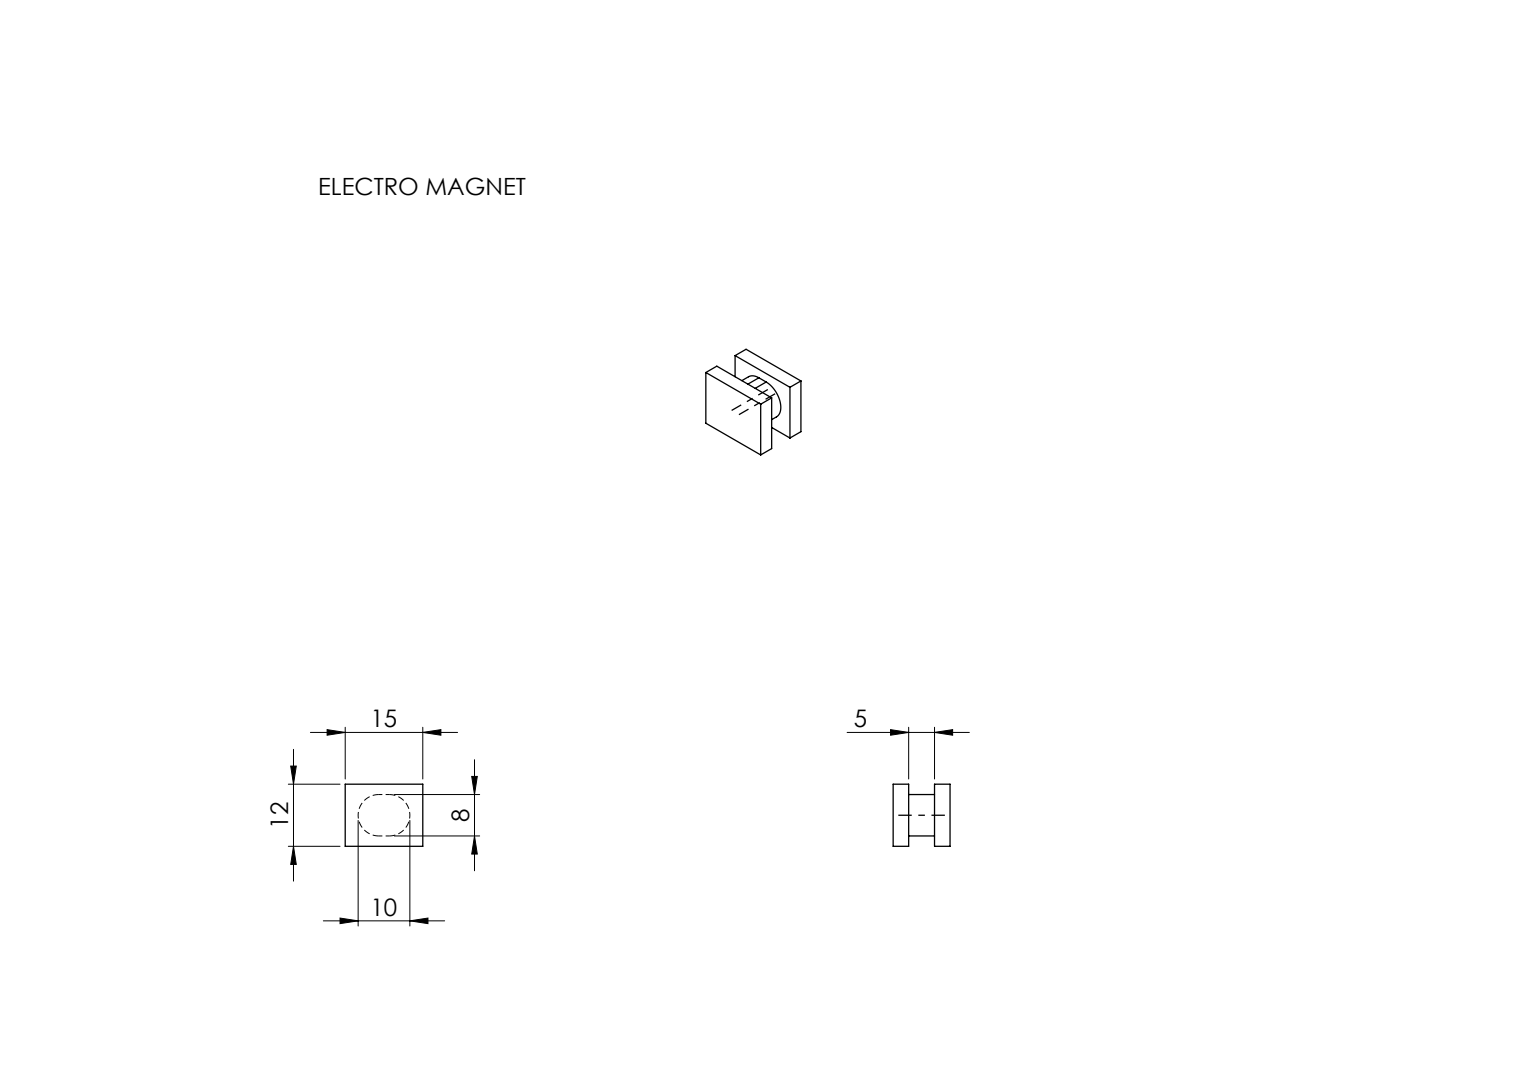
ISO-10303-21;
HEADER;
FILE_DESCRIPTION (('STEP AP214'),
    '1' );
FILE_NAME ('electro magnet.step',
    '2026-10-08T14:41:38',
    ( '' ),
    ( '' ),
    'SwSTEP 2.0',
    'SolidWorks 2026',
    '' );
FILE_SCHEMA (( 'AUTOMOTIVE_DESIGN' ));
ENDSEC;

DATA;
#101=ORIENTED_EDGE ( 'NONE', *, *, #16409, .T. ) ;
#145=VECTOR ( 'NONE', #11392, 1000.000000000000000 ) ;
#171=( NAMED_UNIT ( * ) SI_UNIT ( $, .STERADIAN. ) SOLID_ANGLE_UNIT ( ) );
#187=LINE ( 'NONE', #12134, #5316 ) ;
#194=FACE_OUTER_BOUND ( 'NONE', #3643, .T. ) ;
#207=CIRCLE ( 'NONE', #14282, 4.000000000000001776 ) ;
#299=AXIS2_PLACEMENT_3D ( 'NONE', #12287, #10903, #18180 ) ;
#302=ADVANCED_FACE ( 'NONE', ( #4804 ), #6459, .T. ) ;
#408=LINE ( 'NONE', #5209, #9039 ) ;
#421=UNCERTAINTY_MEASURE_WITH_UNIT (LENGTH_MEASURE( 1.000000000000000082E-05 ), #7921, 'distance_accuracy_value', 'NONE');
#477=EDGE_CURVE ( 'NONE', #3996, #8594, #18791, .T. ) ;
#486=VECTOR ( 'NONE', #10587, 1000.000000000000000 ) ;
#516=VECTOR ( 'NONE', #18188, 1000.000000000000000 ) ;
#549=SURFACE_STYLE_FILL_AREA ( #12311 ) ;
#556=ORIENTED_EDGE ( 'NONE', *, *, #4978, .F. ) ;
#594=CIRCLE ( 'NONE', #10600, 4.000000000000001776 ) ;
#694=ORIENTED_EDGE ( 'NONE', *, *, #13084, .T. ) ;
#703=AXIS2_PLACEMENT_3D ( 'NONE', #5641, #5740, #11602 ) ;
#724=PLANE ( 'NONE',  #16794 ) ;
#781=ADVANCED_FACE ( 'NONE', ( #18300 ), #17023, .F. ) ;
#858=ORIENTED_EDGE ( 'NONE', *, *, #9631, .T. ) ;
#920=CARTESIAN_POINT ( 'NONE',  ( -0.9999999999999945599, -28.00000000000000000, 9.500000000000001776 ) ) ;
#936=AXIS2_PLACEMENT_3D ( 'NONE', #14392, #3821, #15873 ) ;
#1085=ORIENTED_EDGE ( 'NONE', *, *, #13084, .F. ) ;
#1145=ORIENTED_EDGE ( 'NONE', *, *, #7309, .F. ) ;
#1159=LINE ( 'NONE', #17905, #8587 ) ;
#1304=ORIENTED_EDGE ( 'NONE', *, *, #4606, .F. ) ;
#1306=VECTOR ( 'NONE', #7410, 1000.000000000000000 ) ;
#1365=PLANE ( 'NONE',  #2180 ) ;
#1395=CARTESIAN_POINT ( 'NONE',  ( -0.9999999999999945599, -32.00000000000000000, 4.500000000000000888 ) ) ;
#1406=LINE ( 'NONE', #6021, #14690 ) ;
#1438=DIRECTION ( 'NONE',  ( 2.312964634635742957E-16, -1.000000000000000000, 0.000000000000000000 ) ) ;
#1483=ORIENTED_EDGE ( 'NONE', *, *, #18646, .T. ) ;
#1497=DIRECTION ( 'NONE',  ( -1.000000000000000000, 0.000000000000000000, 0.000000000000000000 ) ) ;
#1502=ADVANCED_FACE ( 'NONE', ( #11641 ), #1365, .F. ) ;
#1513=DIRECTION ( 'NONE',  ( -0.000000000000000000, -0.000000000000000000, -1.000000000000000000 ) ) ;
#1536=CARTESIAN_POINT ( 'NONE',  ( -0.9999999999999945599, -28.00000000000000000, 9.500000000000001776 ) ) ;
#1537=DIRECTION ( 'NONE',  ( -0.000000000000000000, -0.000000000000000000, -1.000000000000000000 ) ) ;
#1592=CARTESIAN_POINT ( 'NONE',  ( -0.9999999999999945599, -28.00000000000000000, 9.500000000000001776 ) ) ;
#1613=VECTOR ( 'NONE', #1909, 1000.000000000000000 ) ;
#1632=EDGE_CURVE ( 'NONE', #10157, #8595, #9199, .T. ) ;
#1643=CARTESIAN_POINT ( 'NONE',  ( 7.500000000000005329, -38.00000000000000000, 9.500000000000001776 ) ) ;
#1698=CARTESIAN_POINT ( 'NONE',  ( 1.000000000000000222, -28.00000000000000000, 9.500000000000001776 ) ) ;
#1719=EDGE_CURVE ( 'NONE', #7260, #9088, #15187, .T. ) ;
#1757=DIRECTION ( 'NONE',  ( -1.000000000000000000, 0.000000000000000000, 0.000000000000000000 ) ) ;
#1761=EDGE_CURVE ( 'NONE', #16018, #13407, #187, .T. ) ;
#1781=DIRECTION ( 'NONE',  ( 0.000000000000000000, -1.000000000000000000, 0.000000000000000000 ) ) ;
#1791=AXIS2_PLACEMENT_3D ( 'NONE', #13713, #4815, #7646 ) ;
#1807=CARTESIAN_POINT ( 'NONE',  ( 7.500000000000005329, -26.00000000000000000, 12.50000000000000000 ) ) ;
#1820=EDGE_CURVE ( 'NONE', #6791, #1960, #10951, .T. ) ;
#1857=EDGE_LOOP ( 'NONE', ( #12020, #9397, #15224, #9214 ) ) ;
#1909=DIRECTION ( 'NONE',  ( -0.000000000000000000, -0.000000000000000000, -1.000000000000000000 ) ) ;
#1960=VERTEX_POINT ( 'NONE', #3801 ) ;
#2012=DIRECTION ( 'NONE',  ( -1.000000000000000000, -2.312964634635742957E-16, 0.000000000000000000 ) ) ;
#2145=ORIENTED_EDGE ( 'NONE', *, *, #1820, .F. ) ;
#2180=AXIS2_PLACEMENT_3D ( 'NONE', #8702, #9970, #15972 ) ;
#2370=AXIS2_PLACEMENT_3D ( 'NONE', #8705, #13017, #9888 ) ;
#2375=CARTESIAN_POINT ( 'NONE',  ( 1.000000000000001332, -36.00000000000000711, 4.500000000000000888 ) ) ;
#2397=ADVANCED_FACE ( 'NONE', ( #5068 ), #3299, .F. ) ;
#2504=CARTESIAN_POINT ( 'NONE',  ( 7.500000000000005329, -38.00000000000000000, 4.500000000000000888 ) ) ;
#2546=VECTOR ( 'NONE', #1781, 1000.000000000000000 ) ;
#2553=ORIENTED_EDGE ( 'NONE', *, *, #18646, .F. ) ;
#2695=CIRCLE ( 'NONE', #18053, 4.000000000000001776 ) ;
#2770=FACE_OUTER_BOUND ( 'NONE', #13066, .T. ) ;
#2903=CARTESIAN_POINT ( 'NONE',  ( 7.500000000000005329, -26.00000000000000000, 12.50000000000000000 ) ) ;
#2954=DIRECTION ( 'NONE',  ( -0.000000000000000000, -0.000000000000000000, -1.000000000000000000 ) ) ;
#2987=DIRECTION ( 'NONE',  ( -0.000000000000000000, -0.000000000000000000, -1.000000000000000000 ) ) ;
#3004=VECTOR ( 'NONE', #4487, 1000.000000000000000 ) ;
#3066=VERTEX_POINT ( 'NONE', #15868 ) ;
#3093=DIRECTION ( 'NONE',  ( 0.000000000000000000, -0.000000000000000000, -1.000000000000000000 ) ) ;
#3134=ORIENTED_EDGE ( 'NONE', *, *, #15716, .T. ) ;
#3138=LINE ( 'NONE', #14011, #12507 ) ;
#3168=EDGE_LOOP ( 'NONE', ( #11221, #15374, #4325, #14700 ) ) ;
#3210=SURFACE_STYLE_USAGE ( .BOTH. , #13686 ) ;
#3228=FACE_OUTER_BOUND ( 'NONE', #8260, .T. ) ;
#3299=PLANE ( 'NONE',  #14340 ) ;
#3319=ORIENTED_EDGE ( 'NONE', *, *, #4999, .F. ) ;
#3418=EDGE_CURVE ( 'NONE', #4550, #8057, #11780, .T. ) ;
#3419=DIRECTION ( 'NONE',  ( 0.000000000000000000, 1.000000000000000000, -0.000000000000000000 ) ) ;
#3467=FACE_OUTER_BOUND ( 'NONE', #17184, .T. ) ;
#3512=ORIENTED_EDGE ( 'NONE', *, *, #10326, .F. ) ;
#3516=DIRECTION ( 'NONE',  ( -0.000000000000000000, -0.000000000000000000, -1.000000000000000000 ) ) ;
#3583=DIRECTION ( 'NONE',  ( 0.000000000000000000, 1.000000000000000000, 0.000000000000000000 ) ) ;
#3585=( NAMED_UNIT ( * ) SI_UNIT ( $, .STERADIAN. ) SOLID_ANGLE_UNIT ( ) );
#3620=ORIENTED_EDGE ( 'NONE', *, *, #9152, .T. ) ;
#3643=EDGE_LOOP ( 'NONE', ( #7791, #3319, #1304, #15009 ) ) ;
#3801=CARTESIAN_POINT ( 'NONE',  ( 7.500000000000005329, -38.00000000000000000, 9.500000000000001776 ) ) ;
#3821=DIRECTION ( 'NONE',  ( 0.000000000000000000, 0.000000000000000000, 1.000000000000000000 ) ) ;
#3830=CARTESIAN_POINT ( 'NONE',  ( 7.500000000000005329, -26.00000000000000000, 9.500000000000001776 ) ) ;
#3996=VERTEX_POINT ( 'NONE', #10683 ) ;
#4016=ORIENTED_EDGE ( 'NONE', *, *, #1632, .F. ) ;
#4029=EDGE_CURVE ( 'NONE', #6116, #3066, #10772, .T. ) ;
#4099=CIRCLE ( 'NONE', #8479, 4.000000000000001776 ) ;
#4143=DIRECTION ( 'NONE',  ( -1.000000000000000000, -0.000000000000000000, -0.000000000000000000 ) ) ;
#4193=ORIENTED_EDGE ( 'NONE', *, *, #4980, .T. ) ;
#4287=LINE ( 'NONE', #16045, #3004 ) ;
#4297=DIRECTION ( 'NONE',  ( 0.000000000000000000, -0.000000000000000000, 1.000000000000000000 ) ) ;
#4325=ORIENTED_EDGE ( 'NONE', *, *, #9152, .F. ) ;
#4341=UNCERTAINTY_MEASURE_WITH_UNIT (LENGTH_MEASURE( 1.000000000000000082E-05 ), #4793, 'distance_accuracy_value', 'NONE');
#4347=CARTESIAN_POINT ( 'NONE',  ( -7.499999999999994671, -38.00000000000000000, 4.500000000000000888 ) ) ;
#4417=VECTOR ( 'NONE', #15037, 1000.000000000000000 ) ;
#4484=LINE ( 'NONE', #1643, #5058 ) ;
#4487=DIRECTION ( 'NONE',  ( -0.000000000000000000, -0.000000000000000000, -1.000000000000000000 ) ) ;
#4537=VECTOR ( 'NONE', #6993, 1000.000000000000000 ) ;
#4550=VERTEX_POINT ( 'NONE', #13696 ) ;
#4606=EDGE_CURVE ( 'NONE', #4550, #3996, #12892, .T. ) ;
#4642=DIRECTION ( 'NONE',  ( 0.000000000000000000, 0.000000000000000000, 1.000000000000000000 ) ) ;
#4676=DIRECTION ( 'NONE',  ( 0.000000000000000000, 1.000000000000000000, 0.000000000000000000 ) ) ;
#4677=LINE ( 'NONE', #2903, #12097 ) ;
#4736=CARTESIAN_POINT ( 'NONE',  ( -0.9999999999999945599, -28.00000000000000000, 4.500000000000000888 ) ) ;
#4754=ORIENTED_EDGE ( 'NONE', *, *, #15964, .F. ) ;
#4780=DIRECTION ( 'NONE',  ( 1.000000000000000000, 2.312964634635742957E-16, 0.000000000000000000 ) ) ;
#4793=( LENGTH_UNIT ( ) NAMED_UNIT ( * ) SI_UNIT ( .MILLI., .METRE. ) );
#4804=FACE_OUTER_BOUND ( 'NONE', #13698, .T. ) ;
#4815=DIRECTION ( 'NONE',  ( 0.000000000000000000, 0.000000000000000000, 1.000000000000000000 ) ) ;
#4856=CARTESIAN_POINT ( 'NONE',  ( -0.9999999999999945599, -36.00000000000000711, 9.500000000000001776 ) ) ;
#4861=VECTOR ( 'NONE', #6043, 1000.000000000000000 ) ;
#4937=DIRECTION ( 'NONE',  ( 1.000000000000000000, 0.000000000000000000, 0.000000000000000000 ) ) ;
#4949=FACE_BOUND ( 'NONE', #8943, .T. ) ;
#4978=EDGE_CURVE ( 'NONE', #8057, #16018, #408, .T. ) ;
#4980=EDGE_CURVE ( 'NONE', #3066, #10268, #594, .T. ) ;
#4999=EDGE_CURVE ( 'NONE', #3996, #16018, #18552, .T. ) ;
#5058=VECTOR ( 'NONE', #17914, 1000.000000000000000 ) ;
#5068=FACE_OUTER_BOUND ( 'NONE', #10560, .T. ) ;
#5071=SURFACE_SIDE_STYLE ('',( #549 ) ) ;
#5100=ORIENTED_EDGE ( 'NONE', *, *, #13421, .T. ) ;
#5175=DIRECTION ( 'NONE',  ( 1.000000000000000000, -0.000000000000000000, -0.000000000000000000 ) ) ;
#5179=CARTESIAN_POINT ( 'NONE',  ( -7.499999999999994671, -38.00000000000000000, 9.500000000000001776 ) ) ;
#5209=CARTESIAN_POINT ( 'NONE',  ( 7.500000000000005329, -38.00000000000000000, 1.500000000000000000 ) ) ;
#5256=FILL_AREA_STYLE_COLOUR ( '', #6784 ) ;
#5286=ORIENTED_EDGE ( 'NONE', *, *, #1820, .T. ) ;
#5292=ORIENTED_EDGE ( 'NONE', *, *, #7515, .F. ) ;
#5316=VECTOR ( 'NONE', #13700, 1000.000000000000000 ) ;
#5340=LINE ( 'NONE', #11587, #4537 ) ;
#5366=DIRECTION ( 'NONE',  ( 0.000000000000000000, 1.000000000000000000, 0.000000000000000000 ) ) ;
#5399=DIRECTION ( 'NONE',  ( -0.000000000000000000, -1.000000000000000000, -0.000000000000000000 ) ) ;
#5641=CARTESIAN_POINT ( 'NONE',  ( 0.000000000000000000, 0.000000000000000000, 4.500000000000000888 ) ) ;
#5740=DIRECTION ( 'NONE',  ( 0.000000000000000000, -0.000000000000000000, 1.000000000000000000 ) ) ;
#5768=ORIENTED_EDGE ( 'NONE', *, *, #14263, .F. ) ;
#5776=FACE_OUTER_BOUND ( 'NONE', #3168, .T. ) ;
#5801=PRODUCT_CONTEXT ( 'NONE', #9697, 'mechanical' ) ;
#5824=DIRECTION ( 'NONE',  ( -0.000000000000000000, -0.000000000000000000, -1.000000000000000000 ) ) ;
#5829=PRODUCT_DEFINITION_SHAPE ( 'NONE', 'NONE',  #16256 ) ;
#5848=CARTESIAN_POINT ( 'NONE',  ( -7.499999999999994671, -38.00000000000000000, 12.50000000000000000 ) ) ;
#5973=DIRECTION ( 'NONE',  ( -0.000000000000000000, -0.000000000000000000, -1.000000000000000000 ) ) ;
#6021=CARTESIAN_POINT ( 'NONE',  ( -7.499999999999994671, -26.00000000000000355, 9.500000000000001776 ) ) ;
#6043=DIRECTION ( 'NONE',  ( -1.000000000000000000, -2.312964634635742957E-16, 0.000000000000000000 ) ) ;
#6055=EDGE_CURVE ( 'NONE', #13407, #9088, #3138, .T. ) ;
#6116=VERTEX_POINT ( 'NONE', #9842 ) ;
#6117=DIRECTION ( 'NONE',  ( 0.000000000000000000, -0.000000000000000000, 1.000000000000000000 ) ) ;
#6153=ORIENTED_EDGE ( 'NONE', *, *, #7072, .F. ) ;
#6155=( NAMED_UNIT ( * ) PLANE_ANGLE_UNIT ( ) SI_UNIT ( $, .RADIAN. ) );
#6179=ADVANCED_FACE ( 'NONE', ( #2770 ), #7287, .F. ) ;
#6181=ORIENTED_EDGE ( 'NONE', *, *, #1761, .F. ) ;
#6195=DIRECTION ( 'NONE',  ( 1.000000000000000000, 0.000000000000000000, 0.000000000000000000 ) ) ;
#6201=LINE ( 'NONE', #7361, #486 ) ;
#6292=CARTESIAN_POINT ( 'NONE',  ( 7.500000000000005329, -26.00000000000000000, 4.500000000000000888 ) ) ;
#6314=VECTOR ( 'NONE', #4143, 1000.000000000000000 ) ;
#6324=CARTESIAN_POINT ( 'NONE',  ( -0.9999999999999945599, -36.00000000000000711, 4.500000000000000888 ) ) ;
#6328=UNCERTAINTY_MEASURE_WITH_UNIT (LENGTH_MEASURE( 1.000000000000000082E-05 ), #18306, 'distance_accuracy_value', 'NONE');
#6349=CLOSED_SHELL ( 'NONE', ( #17179, #14773, #17898, #14461, #9964, #10792, #11208, #6407, #6179, #302, #8220, #13820, #9503, #781, #1502, #2397, #18291 ) ) ;
#6354=FILL_AREA_STYLE_COLOUR ( '', #16103 ) ;
#6370=CARTESIAN_POINT ( 'NONE',  ( -0.9999999999999945599, -32.00000000000000000, 9.500000000000001776 ) ) ;
#6407=ADVANCED_FACE ( 'NONE', ( #13950 ), #9334, .T. ) ;
#6421=CARTESIAN_POINT ( 'NONE',  ( -7.499999999999994671, -26.00000000000000355, 12.50000000000000000 ) ) ;
#6422=CARTESIAN_POINT ( 'NONE',  ( -4.999999999999996447, -32.00000000000000000, 4.500000000000000888 ) ) ;
#6459=CYLINDRICAL_SURFACE ( 'NONE', #17272, 4.000000000000001776 ) ;
#6532=CARTESIAN_POINT ( 'NONE',  ( -7.499999999999994671, -38.00000000000000000, 12.50000000000000000 ) ) ;
#6568=VECTOR ( 'NONE', #7836, 1000.000000000000000 ) ;
#6618=ORIENTED_EDGE ( 'NONE', *, *, #11880, .F. ) ;
#6698=VERTEX_POINT ( 'NONE', #13234 ) ;
#6740=DIRECTION ( 'NONE',  ( 0.000000000000000000, 0.000000000000000000, 1.000000000000000000 ) ) ;
#6750=EDGE_LOOP ( 'NONE', ( #7814, #10770, #16833, #12425 ) ) ;
#6784=COLOUR_RGB ( '', 0.66274510, 0.83137255, 0.94901961) ;
#6791=VERTEX_POINT ( 'NONE', #7763 ) ;
#6796=MECHANICAL_DESIGN_GEOMETRIC_PRESENTATION_REPRESENTATION('',(#17732),#17748);
#6899=CARTESIAN_POINT ( 'NONE',  ( 7.500000000000005329, -26.00000000000000000, 1.500000000000000000 ) ) ;
#6941=CARTESIAN_POINT ( 'NONE',  ( 0.000000000000000000, 0.000000000000000000, 1.500000000000000000 ) ) ;
#6993=DIRECTION ( 'NONE',  ( 1.000000000000000000, 0.000000000000000000, 0.000000000000000000 ) ) ;
#6996=LINE ( 'NONE', #920, #15048 ) ;
#7009=FACE_OUTER_BOUND ( 'NONE', #12217, .T. ) ;
#7045=LINE ( 'NONE', #18826, #13144 ) ;
#7070=CARTESIAN_POINT ( 'NONE',  ( -0.9999999999999945599, -28.00000000000000000, 9.500000000000001776 ) ) ;
#7072=EDGE_CURVE ( 'NONE', #8851, #8886, #6996, .T. ) ;
#7107=FACE_BOUND ( 'NONE', #10188, .T. ) ;
#7146=ORIENTED_EDGE ( 'NONE', *, *, #12750, .F. ) ;
#7161=ORIENTED_EDGE ( 'NONE', *, *, #10010, .T. ) ;
#7165=DIRECTION ( 'NONE',  ( 0.000000000000000000, 0.000000000000000000, 1.000000000000000000 ) ) ;
#7183=DIRECTION ( 'NONE',  ( 0.000000000000000000, 1.000000000000000000, 0.000000000000000000 ) ) ;
#7213=FACE_OUTER_BOUND ( 'NONE', #12120, .T. ) ;
#7260=VERTEX_POINT ( 'NONE', #18182 ) ;
#7287=PLANE ( 'NONE',  #15329 ) ;
#7309=EDGE_CURVE ( 'NONE', #3066, #7522, #16707, .T. ) ;
#7361=CARTESIAN_POINT ( 'NONE',  ( -0.9999999999999945599, -28.00000000000000000, 4.500000000000000888 ) ) ;
#7382=DIRECTION ( 'NONE',  ( 0.000000000000000000, -1.000000000000000000, 0.000000000000000000 ) ) ;
#7410=DIRECTION ( 'NONE',  ( 1.000000000000000000, 0.000000000000000000, 0.000000000000000000 ) ) ;
#7424=CARTESIAN_POINT ( 'NONE',  ( 7.500000000000005329, -38.00000000000000000, 4.500000000000000888 ) ) ;
#7515=EDGE_CURVE ( 'NONE', #7522, #8981, #4099, .T. ) ;
#7522=VERTEX_POINT ( 'NONE', #2375 ) ;
#7543=ORIENTED_EDGE ( 'NONE', *, *, #7625, .F. ) ;
#7625=EDGE_CURVE ( 'NONE', #10268, #8851, #10191, .T. ) ;
#7646=DIRECTION ( 'NONE',  ( 1.000000000000000000, 0.000000000000000000, 0.000000000000000000 ) ) ;
#7678=DIRECTION ( 'NONE',  ( -0.000000000000000000, -0.000000000000000000, -1.000000000000000000 ) ) ;
#7763=CARTESIAN_POINT ( 'NONE',  ( -7.499999999999994671, -38.00000000000000000, 9.500000000000001776 ) ) ;
#7791=ORIENTED_EDGE ( 'NONE', *, *, #4978, .T. ) ;
#7799=LINE ( 'NONE', #16423, #4861 ) ;
#7814=ORIENTED_EDGE ( 'NONE', *, *, #6055, .T. ) ;
#7836=DIRECTION ( 'NONE',  ( 1.000000000000000000, 0.000000000000000000, 0.000000000000000000 ) ) ;
#7921=( LENGTH_UNIT ( ) NAMED_UNIT ( * ) SI_UNIT ( .MILLI., .METRE. ) );
#7939=DIRECTION ( 'NONE',  ( 1.000000000000000000, 0.000000000000000000, 0.000000000000000000 ) ) ;
#7941=DIRECTION ( 'NONE',  ( 0.000000000000000000, 0.000000000000000000, 1.000000000000000000 ) ) ;
#7996=VECTOR ( 'NONE', #2012, 1000.000000000000000 ) ;
#8057=VERTEX_POINT ( 'NONE', #18615 ) ;
#8205=VECTOR ( 'NONE', #4676, 1000.000000000000000 ) ;
#8220=ADVANCED_FACE ( 'NONE', ( #7213 ), #9075, .F. ) ;
#8254=EDGE_CURVE ( 'NONE', #15143, #13986, #10436, .T. ) ;
#8255=ORIENTED_EDGE ( 'NONE', *, *, #4029, .F. ) ;
#8260=EDGE_LOOP ( 'NONE', ( #7161, #17171, #11662, #12090 ) ) ;
#8398=EDGE_CURVE ( 'NONE', #13986, #10157, #16928, .T. ) ;
#8439=ORIENTED_EDGE ( 'NONE', *, *, #11905, .F. ) ;
#8479=AXIS2_PLACEMENT_3D ( 'NONE', #12850, #7165, #14425 ) ;
#8513=ORIENTED_EDGE ( 'NONE', *, *, #11880, .T. ) ;
#8587=VECTOR ( 'NONE', #2987, 1000.000000000000000 ) ;
#8594=VERTEX_POINT ( 'NONE', #12688 ) ;
#8595=VERTEX_POINT ( 'NONE', #17659 ) ;
#8702=CARTESIAN_POINT ( 'NONE',  ( -7.499999999999994671, -26.00000000000000355, 12.50000000000000000 ) ) ;
#8705=CARTESIAN_POINT ( 'NONE',  ( -7.499999999999994671, -38.00000000000000000, 4.500000000000000888 ) ) ;
#8730=CYLINDRICAL_SURFACE ( 'NONE', #11736, 4.000000000000001776 ) ;
#8843=PRODUCT_DEFINITION_CONTEXT ( 'detailed design', #13441, 'design' ) ;
#8851=VERTEX_POINT ( 'NONE', #1592 ) ;
#8886=VERTEX_POINT ( 'NONE', #4736 ) ;
#8889=PLANE ( 'NONE',  #19275 ) ;
#8900=EDGE_LOOP ( 'NONE', ( #19185, #10269, #3512, #12152 ) ) ;
#8905=CARTESIAN_POINT ( 'NONE',  ( 7.500000000000005329, -38.00000000000000000, 12.50000000000000000 ) ) ;
#8943=EDGE_LOOP ( 'NONE', ( #16290, #1483, #858, #18898, #4193 ) ) ;
#8981=VERTEX_POINT ( 'NONE', #17077 ) ;
#9039=VECTOR ( 'NONE', #11165, 1000.000000000000000 ) ;
#9075=PLANE ( 'NONE',  #11609 ) ;
#9088=VERTEX_POINT ( 'NONE', #18360 ) ;
#9152=EDGE_CURVE ( 'NONE', #7260, #4550, #7045, .T. ) ;
#9157=LINE ( 'NONE', #6421, #1613 ) ;
#9199=LINE ( 'NONE', #18127, #14073 ) ;
#9214=ORIENTED_EDGE ( 'NONE', *, *, #15716, .F. ) ;
#9240=AXIS2_PLACEMENT_3D ( 'NONE', #15325, #9628, #18669 ) ;
#9318=CARTESIAN_POINT ( 'NONE',  ( 7.500000000000005329, -38.00000000000000000, 4.500000000000000888 ) ) ;
#9323=CARTESIAN_POINT ( 'NONE',  ( 7.500000000000005329, -38.00000000000000000, 1.500000000000000000 ) ) ;
#9334=CYLINDRICAL_SURFACE ( 'NONE', #299, 4.000000000000001776 ) ;
#9369=( NAMED_UNIT ( * ) PLANE_ANGLE_UNIT ( ) SI_UNIT ( $, .RADIAN. ) );
#9397=ORIENTED_EDGE ( 'NONE', *, *, #15964, .T. ) ;
#9483=DIRECTION ( 'NONE',  ( -1.000000000000000000, 0.000000000000000000, 0.000000000000000000 ) ) ;
#9503=ADVANCED_FACE ( 'NONE', ( #3228 ), #15189, .F. ) ;
#9628=DIRECTION ( 'NONE',  ( 0.000000000000000000, -0.000000000000000000, 1.000000000000000000 ) ) ;
#9631=EDGE_CURVE ( 'NONE', #11032, #6116, #11288, .T. ) ;
#9684=ORIENTED_EDGE ( 'NONE', *, *, #477, .T. ) ;
#9697=APPLICATION_CONTEXT ( 'automotive_design' ) ;
#9737=VECTOR ( 'NONE', #13830, 1000.000000000000000 ) ;
#9840=ORIENTED_EDGE ( 'NONE', *, *, #10010, .F. ) ;
#9842=CARTESIAN_POINT ( 'NONE',  ( -0.9999999999999945599, -36.00000000000000711, 9.500000000000001776 ) ) ;
#9864=ORIENTED_EDGE ( 'NONE', *, *, #18143, .F. ) ;
#9872=FACE_OUTER_BOUND ( 'NONE', #18837, .T. ) ;
#9888=DIRECTION ( 'NONE',  ( 0.000000000000000000, 0.000000000000000000, -1.000000000000000000 ) ) ;
#9897=VECTOR ( 'NONE', #2954, 1000.000000000000000 ) ;
#9964=ADVANCED_FACE ( 'NONE', ( #13279 ), #19376, .F. ) ;
#9970=DIRECTION ( 'NONE',  ( 1.000000000000000000, 0.000000000000000000, -0.000000000000000000 ) ) ;
#9978=ORIENTED_EDGE ( 'NONE', *, *, #13207, .T. ) ;
#10010=EDGE_CURVE ( 'NONE', #1960, #14775, #4484, .T. ) ;
#10089=VERTEX_POINT ( 'NONE', #6324 ) ;
#10101=EDGE_CURVE ( 'NONE', #8595, #6698, #9157, .T. ) ;
#10157=VERTEX_POINT ( 'NONE', #1807 ) ;
#10188=EDGE_LOOP ( 'NONE', ( #18902, #5768, #5292, #11263, #7146 ) ) ;
#10191=LINE ( 'NONE', #7070, #6314 ) ;
#10268=VERTEX_POINT ( 'NONE', #15592 ) ;
#10269=ORIENTED_EDGE ( 'NONE', *, *, #13095, .F. ) ;
#10310=EDGE_CURVE ( 'NONE', #8594, #13407, #10880, .T. ) ;
#10326=EDGE_CURVE ( 'NONE', #8595, #15143, #18551, .T. ) ;
#10436=LINE ( 'NONE', #5848, #1306 ) ;
#10511=CARTESIAN_POINT ( 'NONE',  ( 1.000000000000001332, -36.00000000000000711, 9.500000000000001776 ) ) ;
#10542=DIRECTION ( 'NONE',  ( 0.000000000000000000, -0.000000000000000000, 1.000000000000000000 ) ) ;
#10560=EDGE_LOOP ( 'NONE', ( #5286, #9864, #11648, #14802 ) ) ;
#10569=ORIENTED_EDGE ( 'NONE', *, *, #14263, .T. ) ;
#10587=DIRECTION ( 'NONE',  ( -1.000000000000000000, -0.000000000000000000, -0.000000000000000000 ) ) ;
#10593=FACE_OUTER_BOUND ( 'NONE', #1857, .T. ) ;
#10600=AXIS2_PLACEMENT_3D ( 'NONE', #17163, #10882, #12354 ) ;
#10614=VECTOR ( 'NONE', #12179, 1000.000000000000000 ) ;
#10660=AXIS2_PLACEMENT_3D ( 'NONE', #12008, #1438, #19280 ) ;
#10683=CARTESIAN_POINT ( 'NONE',  ( 7.500000000000005329, -38.00000000000000000, 4.500000000000000888 ) ) ;
#10770=ORIENTED_EDGE ( 'NONE', *, *, #1719, .F. ) ;
#10772=LINE ( 'NONE', #14118, #15059 ) ;
#10792=ADVANCED_FACE ( 'NONE', ( #7107, #7009 ), #14555, .T. ) ;
#10873=DIRECTION ( 'NONE',  ( -1.000000000000000000, -2.312964634635742957E-16, 0.000000000000000000 ) ) ;
#10880=LINE ( 'NONE', #6292, #9737 ) ;
#10882=DIRECTION ( 'NONE',  ( 0.000000000000000000, 0.000000000000000000, 1.000000000000000000 ) ) ;
#10903=DIRECTION ( 'NONE',  ( -0.000000000000000000, -0.000000000000000000, -1.000000000000000000 ) ) ;
#10951=LINE ( 'NONE', #5179, #6568 ) ;
#11032=VERTEX_POINT ( 'NONE', #17061 ) ;
#11098=( GEOMETRIC_REPRESENTATION_CONTEXT ( 3 ) GLOBAL_UNCERTAINTY_ASSIGNED_CONTEXT ( ( #4341 ) ) GLOBAL_UNIT_ASSIGNED_CONTEXT ( ( #4793, #9369, #171 ) ) REPRESENTATION_CONTEXT ( 'NONE', 'WORKASPACE' ) );
#11137=CARTESIAN_POINT ( 'NONE',  ( 7.500000000000005329, -38.00000000000000000, 4.500000000000000888 ) ) ;
#11165=DIRECTION ( 'NONE',  ( 1.000000000000000000, -0.000000000000000000, -0.000000000000000000 ) ) ;
#11188=PLANE ( 'NONE',  #9240 ) ;
#11208=ADVANCED_FACE ( 'NONE', ( #9872 ), #17520, .F. ) ;
#11221=ORIENTED_EDGE ( 'NONE', *, *, #13455, .T. ) ;
#11263=ORIENTED_EDGE ( 'NONE', *, *, #13421, .F. ) ;
#11288=CIRCLE ( 'NONE', #17566, 4.000000000000001776 ) ;
#11392=DIRECTION ( 'NONE',  ( -0.000000000000000000, -1.000000000000000000, -0.000000000000000000 ) ) ;
#11413=PRODUCT_DEFINITION_FORMATION_WITH_SPECIFIED_SOURCE ( 'ANY', '', #11758, .NOT_KNOWN. ) ;
#11468=CARTESIAN_POINT ( 'NONE',  ( 7.500000000000005329, -38.00000000000000000, 12.50000000000000000 ) ) ;
#11587=CARTESIAN_POINT ( 'NONE',  ( -0.9999999999999945599, -36.00000000000000711, 4.500000000000000888 ) ) ;
#11602=DIRECTION ( 'NONE',  ( 1.000000000000000000, 0.000000000000000000, -0.000000000000000000 ) ) ;
#11609=AXIS2_PLACEMENT_3D ( 'NONE', #1536, #17607, #3093 ) ;
#11641=FACE_OUTER_BOUND ( 'NONE', #8900, .T. ) ;
#11648=ORIENTED_EDGE ( 'NONE', *, *, #8254, .F. ) ;
#11662=ORIENTED_EDGE ( 'NONE', *, *, #8398, .F. ) ;
#11736=AXIS2_PLACEMENT_3D ( 'NONE', #14924, #16589, #1497 ) ;
#11758=PRODUCT ( 'electro magnet', 'electro magnet', '', ( #5801 ) ) ;
#11763=SHAPE_DEFINITION_REPRESENTATION ( #5829, #15417 ) ;
#11780=LINE ( 'NONE', #4347, #18501 ) ;
#11783=ORIENTED_EDGE ( 'NONE', *, *, #6055, .F. ) ;
#11820=ORIENTED_EDGE ( 'NONE', *, *, #1632, .T. ) ;
#11834=DIRECTION ( 'NONE',  ( -1.000000000000000000, -2.312964634635742957E-16, 0.000000000000000000 ) ) ;
#11870=DIRECTION ( 'NONE',  ( 1.000000000000000000, 0.000000000000000000, 0.000000000000000000 ) ) ;
#11880=EDGE_CURVE ( 'NONE', #10268, #8981, #14937, .T. ) ;
#11905=EDGE_CURVE ( 'NONE', #6698, #6791, #1406, .T. ) ;
#11920=AXIS2_PLACEMENT_3D ( 'NONE', #8905, #1757, #16257 ) ;
#12008=CARTESIAN_POINT ( 'NONE',  ( 7.500000000000005329, -26.00000000000000000, 4.500000000000000888 ) ) ;
#12020=ORIENTED_EDGE ( 'NONE', *, *, #9631, .F. ) ;
#12023=DIRECTION ( 'NONE',  ( 0.000000000000000000, 0.000000000000000000, 1.000000000000000000 ) ) ;
#12069=CARTESIAN_POINT ( 'NONE',  ( -0.9999999999999945599, -32.00000000000000000, 9.500000000000001776 ) ) ;
#12090=ORIENTED_EDGE ( 'NONE', *, *, #18143, .T. ) ;
#12097=VECTOR ( 'NONE', #1537, 1000.000000000000000 ) ;
#12117=( NAMED_UNIT ( * ) SI_UNIT ( $, .STERADIAN. ) SOLID_ANGLE_UNIT ( ) );
#12120=EDGE_LOOP ( 'NONE', ( #10569, #6153, #7543, #8513 ) ) ;
#12122=FACE_OUTER_BOUND ( 'NONE', #16342, .T. ) ;
#12134=CARTESIAN_POINT ( 'NONE',  ( 7.500000000000005329, -38.00000000000000000, 1.500000000000000000 ) ) ;
#12152=ORIENTED_EDGE ( 'NONE', *, *, #10101, .T. ) ;
#12176=AXIS2_PLACEMENT_3D ( 'NONE', #13672, #18400, #4780 ) ;
#12179=DIRECTION ( 'NONE',  ( -0.000000000000000000, -0.000000000000000000, -1.000000000000000000 ) ) ;
#12217=EDGE_LOOP ( 'NONE', ( #3620, #16605, #9684, #9978 ) ) ;
#12246=ORIENTED_EDGE ( 'NONE', *, *, #7309, .T. ) ;
#12287=CARTESIAN_POINT ( 'NONE',  ( -0.9999999999999945599, -32.00000000000000000, 9.500000000000001776 ) ) ;
#12311=FILL_AREA_STYLE ('',( #5256 ) ) ;
#12317=SURFACE_STYLE_FILL_AREA ( #16739 ) ;
#12334=PLANE ( 'NONE',  #17100 ) ;
#12354=DIRECTION ( 'NONE',  ( 1.000000000000000000, 0.000000000000000000, 0.000000000000000000 ) ) ;
#12407=SURFACE_STYLE_USAGE ( .BOTH. , #5071 ) ;
#12425=ORIENTED_EDGE ( 'NONE', *, *, #10310, .T. ) ;
#12427=CARTESIAN_POINT ( 'NONE',  ( 1.000000000000001998, -32.00000000000000000, 9.500000000000001776 ) ) ;
#12499=CARTESIAN_POINT ( 'NONE',  ( 7.500000000000005329, -38.00000000000000000, 12.50000000000000000 ) ) ;
#12501=( NAMED_UNIT ( * ) PLANE_ANGLE_UNIT ( ) SI_UNIT ( $, .RADIAN. ) );
#12507=VECTOR ( 'NONE', #10873, 1000.000000000000000 ) ;
#12585=DIRECTION ( 'NONE',  ( 1.000000000000000000, 0.000000000000000000, -0.000000000000000000 ) ) ;
#12688=CARTESIAN_POINT ( 'NONE',  ( 7.500000000000005329, -26.00000000000000000, 4.500000000000000888 ) ) ;
#12750=EDGE_CURVE ( 'NONE', #15578, #10089, #13460, .T. ) ;
#12850=CARTESIAN_POINT ( 'NONE',  ( 1.000000000000001998, -32.00000000000000000, 4.500000000000000888 ) ) ;
#12892=LINE ( 'NONE', #11137, #16559 ) ;
#12955=MECHANICAL_DESIGN_GEOMETRIC_PRESENTATION_REPRESENTATION('',(#13275),#17989);
#13017=DIRECTION ( 'NONE',  ( 1.000000000000000000, 0.000000000000000000, 0.000000000000000000 ) ) ;
#13066=EDGE_LOOP ( 'NONE', ( #5100, #1145, #8255, #3134 ) ) ;
#13084=EDGE_CURVE ( 'NONE', #14775, #6698, #7799, .T. ) ;
#13090=VECTOR ( 'NONE', #1513, 1000.000000000000000 ) ;
#13095=EDGE_CURVE ( 'NONE', #15143, #6791, #1159, .T. ) ;
#13144=VECTOR ( 'NONE', #5399, 1000.000000000000000 ) ;
#13207=EDGE_CURVE ( 'NONE', #8594, #7260, #14252, .T. ) ;
#13234=CARTESIAN_POINT ( 'NONE',  ( -7.499999999999994671, -26.00000000000000355, 9.500000000000001776 ) ) ;
#13250=ORIENTED_EDGE ( 'NONE', *, *, #10326, .T. ) ;
#13275=STYLED_ITEM ( 'NONE', ( #18313 ), #18799 ) ;
#13279=FACE_OUTER_BOUND ( 'NONE', #6750, .T. ) ;
#13407=VERTEX_POINT ( 'NONE', #6899 ) ;
#13421=EDGE_CURVE ( 'NONE', #10089, #7522, #5340, .T. ) ;
#13430=VECTOR ( 'NONE', #5973, 1000.000000000000000 ) ;
#13441=APPLICATION_CONTEXT ( 'automotive_design' ) ;
#13455=EDGE_CURVE ( 'NONE', #9088, #8057, #18959, .T. ) ;
#13460=CIRCLE ( 'NONE', #936, 4.000000000000001776 ) ;
#13615=ORIENTED_EDGE ( 'NONE', *, *, #7515, .T. ) ;
#13672=CARTESIAN_POINT ( 'NONE',  ( 7.500000000000005329, -26.00000000000000000, 12.50000000000000000 ) ) ;
#13682=FACE_OUTER_BOUND ( 'NONE', #14884, .T. ) ;
#13686=SURFACE_SIDE_STYLE ('',( #12317 ) ) ;
#13696=CARTESIAN_POINT ( 'NONE',  ( -7.499999999999994671, -38.00000000000000000, 4.500000000000000888 ) ) ;
#13698=EDGE_LOOP ( 'NONE', ( #13615, #6618, #18468, #12246 ) ) ;
#13700=DIRECTION ( 'NONE',  ( 0.000000000000000000, 1.000000000000000000, 0.000000000000000000 ) ) ;
#13713=CARTESIAN_POINT ( 'NONE',  ( 0.000000000000000000, 0.000000000000000000, 0.000000000000000000 ) ) ;
#13777=DIRECTION ( 'NONE',  ( 0.000000000000000000, -0.000000000000000000, 1.000000000000000000 ) ) ;
#13820=ADVANCED_FACE ( 'NONE', ( #3467, #4949 ), #11188, .F. ) ;
#13830=DIRECTION ( 'NONE',  ( -0.000000000000000000, -0.000000000000000000, -1.000000000000000000 ) ) ;
#13878=PRESENTATION_STYLE_ASSIGNMENT (( #12407 ) ) ;
#13950=FACE_OUTER_BOUND ( 'NONE', #14196, .T. ) ;
#13986=VERTEX_POINT ( 'NONE', #11468 ) ;
#14011=CARTESIAN_POINT ( 'NONE',  ( 7.500000000000005329, -26.00000000000000000, 1.500000000000000000 ) ) ;
#14013=ORIENTED_EDGE ( 'NONE', *, *, #8398, .T. ) ;
#14019=CARTESIAN_POINT ( 'NONE',  ( -7.499999999999994671, -26.00000000000000355, 12.50000000000000000 ) ) ;
#14073=VECTOR ( 'NONE', #11834, 1000.000000000000000 ) ;
#14118=CARTESIAN_POINT ( 'NONE',  ( -0.9999999999999945599, -36.00000000000000711, 9.500000000000001776 ) ) ;
#14196=EDGE_LOOP ( 'NONE', ( #4754, #2553, #17637, #16667 ) ) ;
#14211=EDGE_LOOP ( 'NONE', ( #694, #17327, #4016, #101 ) ) ;
#14252=LINE ( 'NONE', #18398, #7996 ) ;
#14263=EDGE_CURVE ( 'NONE', #8981, #8886, #6201, .T. ) ;
#14282=AXIS2_PLACEMENT_3D ( 'NONE', #12069, #4642, #11870 ) ;
#14340=AXIS2_PLACEMENT_3D ( 'NONE', #6532, #3583, #13777 ) ;
#14392=CARTESIAN_POINT ( 'NONE',  ( -0.9999999999999945599, -32.00000000000000000, 4.500000000000000888 ) ) ;
#14425=DIRECTION ( 'NONE',  ( 1.000000000000000000, 0.000000000000000000, 0.000000000000000000 ) ) ;
#14461=ADVANCED_FACE ( 'NONE', ( #12122 ), #8889, .F. ) ;
#14555=PLANE ( 'NONE',  #703 ) ;
#14690=VECTOR ( 'NONE', #7382, 1000.000000000000000 ) ;
#14700=ORIENTED_EDGE ( 'NONE', *, *, #1719, .T. ) ;
#14773=ADVANCED_FACE ( 'NONE', ( #5776 ), #16165, .F. ) ;
#14775=VERTEX_POINT ( 'NONE', #3830 ) ;
#14786=DIRECTION ( 'NONE',  ( 1.000000000000000000, 0.000000000000000000, -0.000000000000000000 ) ) ;
#14802=ORIENTED_EDGE ( 'NONE', *, *, #13095, .T. ) ;
#14824=CARTESIAN_POINT ( 'NONE',  ( -4.999999999999996447, -32.00000000000000000, 9.500000000000001776 ) ) ;
#14877=DIRECTION ( 'NONE',  ( -1.000000000000000000, 0.000000000000000000, 0.000000000000000000 ) ) ;
#14884=EDGE_LOOP ( 'NONE', ( #14013, #11820, #13250, #17131 ) ) ;
#14924=CARTESIAN_POINT ( 'NONE',  ( -0.9999999999999945599, -32.00000000000000000, 9.500000000000001776 ) ) ;
#14937=LINE ( 'NONE', #1698, #10614 ) ;
#15009=ORIENTED_EDGE ( 'NONE', *, *, #3418, .T. ) ;
#15037=DIRECTION ( 'NONE',  ( -0.000000000000000000, -0.000000000000000000, -1.000000000000000000 ) ) ;
#15048=VECTOR ( 'NONE', #5824, 1000.000000000000000 ) ;
#15059=VECTOR ( 'NONE', #6195, 1000.000000000000000 ) ;
#15074=VECTOR ( 'NONE', #5366, 1000.000000000000000 ) ;
#15143=VERTEX_POINT ( 'NONE', #15553 ) ;
#15187=LINE ( 'NONE', #16428, #13430 ) ;
#15189=PLANE ( 'NONE',  #11920 ) ;
#15224=ORIENTED_EDGE ( 'NONE', *, *, #12750, .T. ) ;
#15325=CARTESIAN_POINT ( 'NONE',  ( 0.000000000000000000, 0.000000000000000000, 9.500000000000001776 ) ) ;
#15329=AXIS2_PLACEMENT_3D ( 'NONE', #16304, #7183, #6117 ) ;
#15374=ORIENTED_EDGE ( 'NONE', *, *, #3418, .F. ) ;
#15417=SHAPE_REPRESENTATION ( 'electro magnet', ( #1791 ), #11098 ) ;
#15553=CARTESIAN_POINT ( 'NONE',  ( -7.499999999999994671, -38.00000000000000000, 12.50000000000000000 ) ) ;
#15578=VERTEX_POINT ( 'NONE', #6422 ) ;
#15592=CARTESIAN_POINT ( 'NONE',  ( 1.000000000000000222, -28.00000000000000000, 9.500000000000001776 ) ) ;
#15716=EDGE_CURVE ( 'NONE', #6116, #10089, #18085, .T. ) ;
#15868=CARTESIAN_POINT ( 'NONE',  ( 1.000000000000001332, -36.00000000000000711, 9.500000000000001776 ) ) ;
#15873=DIRECTION ( 'NONE',  ( 1.000000000000000000, 0.000000000000000000, 0.000000000000000000 ) ) ;
#15964=EDGE_CURVE ( 'NONE', #11032, #15578, #16787, .T. ) ;
#15972=DIRECTION ( 'NONE',  ( -0.000000000000000000, 0.000000000000000000, -1.000000000000000000 ) ) ;
#16018=VERTEX_POINT ( 'NONE', #9323 ) ;
#16045=CARTESIAN_POINT ( 'NONE',  ( 7.500000000000005329, -38.00000000000000000, 12.50000000000000000 ) ) ;
#16103=COLOUR_RGB ( '', 0.66274510, 0.83137255, 0.94901961) ;
#16165=PLANE ( 'NONE',  #2370 ) ;
#16256=PRODUCT_DEFINITION ( 'UNKNOWN', '', #11413, #8843 ) ;
#16257=DIRECTION ( 'NONE',  ( 0.000000000000000000, 0.000000000000000000, 1.000000000000000000 ) ) ;
#16290=ORIENTED_EDGE ( 'NONE', *, *, #7625, .T. ) ;
#16304=CARTESIAN_POINT ( 'NONE',  ( -0.9999999999999945599, -36.00000000000000711, 9.500000000000001776 ) ) ;
#16342=EDGE_LOOP ( 'NONE', ( #19315, #19391, #17708, #17738 ) ) ;
#16409=EDGE_CURVE ( 'NONE', #10157, #14775, #4677, .T. ) ;
#16423=CARTESIAN_POINT ( 'NONE',  ( 7.500000000000005329, -26.00000000000000000, 9.500000000000001776 ) ) ;
#16428=CARTESIAN_POINT ( 'NONE',  ( -7.499999999999994671, -26.00000000000000355, 4.500000000000000888 ) ) ;
#16536=MANIFOLD_SOLID_BREP ( 'Boss-Extrude3', #6349 ) ;
#16559=VECTOR ( 'NONE', #5175, 1000.000000000000000 ) ;
#16589=DIRECTION ( 'NONE',  ( -0.000000000000000000, -0.000000000000000000, -1.000000000000000000 ) ) ;
#16605=ORIENTED_EDGE ( 'NONE', *, *, #4606, .T. ) ;
#16667=ORIENTED_EDGE ( 'NONE', *, *, #18796, .T. ) ;
#16707=LINE ( 'NONE', #10511, #4417 ) ;
#16739=FILL_AREA_STYLE ('',( #6354 ) ) ;
#16787=LINE ( 'NONE', #14824, #9897 ) ;
#16791=DIRECTION ( 'NONE',  ( 0.000000000000000000, 0.000000000000000000, 1.000000000000000000 ) ) ;
#16794=AXIS2_PLACEMENT_3D ( 'NONE', #18107, #10542, #12585 ) ;
#16833=ORIENTED_EDGE ( 'NONE', *, *, #13207, .F. ) ;
#16928=LINE ( 'NONE', #12499, #8205 ) ;
#17023=PLANE ( 'NONE',  #12176 ) ;
#17061=CARTESIAN_POINT ( 'NONE',  ( -4.999999999999996447, -32.00000000000000000, 9.500000000000001776 ) ) ;
#17077=CARTESIAN_POINT ( 'NONE',  ( 1.000000000000000222, -28.00000000000000000, 4.500000000000000888 ) ) ;
#17100=AXIS2_PLACEMENT_3D ( 'NONE', #18332, #3419, #7941 ) ;
#17131=ORIENTED_EDGE ( 'NONE', *, *, #8254, .T. ) ;
#17163=CARTESIAN_POINT ( 'NONE',  ( 1.000000000000001998, -32.00000000000000000, 9.500000000000001776 ) ) ;
#17171=ORIENTED_EDGE ( 'NONE', *, *, #16409, .F. ) ;
#17179=ADVANCED_FACE ( 'NONE', ( #10593 ), #8730, .T. ) ;
#17184=EDGE_LOOP ( 'NONE', ( #9840, #2145, #8439, #1085 ) ) ;
#17272=AXIS2_PLACEMENT_3D ( 'NONE', #12427, #3516, #9483 ) ;
#17282=AXIS2_PLACEMENT_3D ( 'NONE', #6941, #4297, #14786 ) ;
#17327=ORIENTED_EDGE ( 'NONE', *, *, #10101, .F. ) ;
#17520=PLANE ( 'NONE',  #17282 ) ;
#17566=AXIS2_PLACEMENT_3D ( 'NONE', #6370, #6740, #7939 ) ;
#17607=DIRECTION ( 'NONE',  ( 0.000000000000000000, -1.000000000000000000, 0.000000000000000000 ) ) ;
#17637=ORIENTED_EDGE ( 'NONE', *, *, #7072, .T. ) ;
#17659=CARTESIAN_POINT ( 'NONE',  ( -7.499999999999994671, -26.00000000000000355, 12.50000000000000000 ) ) ;
#17708=ORIENTED_EDGE ( 'NONE', *, *, #477, .F. ) ;
#17732=STYLED_ITEM ( 'NONE', ( #13878 ), #16536 ) ;
#17738=ORIENTED_EDGE ( 'NONE', *, *, #4999, .T. ) ;
#17748=( GEOMETRIC_REPRESENTATION_CONTEXT ( 3 ) GLOBAL_UNCERTAINTY_ASSIGNED_CONTEXT ( ( #6328 ) ) GLOBAL_UNIT_ASSIGNED_CONTEXT ( ( #18306, #12501, #3585 ) ) REPRESENTATION_CONTEXT ( 'NONE', 'WORKASPACE' ) );
#17898=ADVANCED_FACE ( 'NONE', ( #194 ), #12334, .F. ) ;
#17905=CARTESIAN_POINT ( 'NONE',  ( -7.499999999999994671, -38.00000000000000000, 12.50000000000000000 ) ) ;
#17914=DIRECTION ( 'NONE',  ( 0.000000000000000000, 1.000000000000000000, 0.000000000000000000 ) ) ;
#17989=( GEOMETRIC_REPRESENTATION_CONTEXT ( 3 ) GLOBAL_UNCERTAINTY_ASSIGNED_CONTEXT ( ( #421 ) ) GLOBAL_UNIT_ASSIGNED_CONTEXT ( ( #7921, #6155, #12117 ) ) REPRESENTATION_CONTEXT ( 'NONE', 'WORKASPACE' ) );
#18011=ORIENTED_EDGE ( 'NONE', *, *, #13455, .F. ) ;
#18053=AXIS2_PLACEMENT_3D ( 'NONE', #1395, #16791, #4937 ) ;
#18085=LINE ( 'NONE', #4856, #516 ) ;
#18107=CARTESIAN_POINT ( 'NONE',  ( 0.000000000000000000, 0.000000000000000000, 12.50000000000000000 ) ) ;
#18112=SHAPE_REPRESENTATION_RELATIONSHIP ( 'NONE' , 'NONE' ,  #15417, #18799 ) ;
#18127=CARTESIAN_POINT ( 'NONE',  ( 7.500000000000005329, -26.00000000000000000, 12.50000000000000000 ) ) ;
#18143=EDGE_CURVE ( 'NONE', #13986, #1960, #4287, .T. ) ;
#18180=DIRECTION ( 'NONE',  ( -1.000000000000000000, 0.000000000000000000, 0.000000000000000000 ) ) ;
#18182=CARTESIAN_POINT ( 'NONE',  ( -7.499999999999994671, -26.00000000000000355, 4.500000000000000888 ) ) ;
#18188=DIRECTION ( 'NONE',  ( -0.000000000000000000, -0.000000000000000000, -1.000000000000000000 ) ) ;
#18291=ADVANCED_FACE ( 'NONE', ( #13682 ), #724, .T. ) ;
#18300=FACE_OUTER_BOUND ( 'NONE', #14211, .T. ) ;
#18306=( LENGTH_UNIT ( ) NAMED_UNIT ( * ) SI_UNIT ( .MILLI., .METRE. ) );
#18313=PRESENTATION_STYLE_ASSIGNMENT (( #3210 ) ) ;
#18332=CARTESIAN_POINT ( 'NONE',  ( 7.500000000000005329, -38.00000000000000000, 4.500000000000000888 ) ) ;
#18360=CARTESIAN_POINT ( 'NONE',  ( -7.499999999999994671, -26.00000000000000355, 1.500000000000000000 ) ) ;
#18398=CARTESIAN_POINT ( 'NONE',  ( 7.500000000000005329, -26.00000000000000000, 4.500000000000000888 ) ) ;
#18400=DIRECTION ( 'NONE',  ( 2.312964634635742957E-16, -1.000000000000000000, 0.000000000000000000 ) ) ;
#18468=ORIENTED_EDGE ( 'NONE', *, *, #4980, .F. ) ;
#18501=VECTOR ( 'NONE', #7678, 1000.000000000000000 ) ;
#18551=LINE ( 'NONE', #14019, #2546 ) ;
#18552=LINE ( 'NONE', #9318, #13090 ) ;
#18615=CARTESIAN_POINT ( 'NONE',  ( -7.499999999999994671, -38.00000000000000000, 1.500000000000000000 ) ) ;
#18646=EDGE_CURVE ( 'NONE', #8851, #11032, #207, .T. ) ;
#18669=DIRECTION ( 'NONE',  ( 1.000000000000000000, 0.000000000000000000, -0.000000000000000000 ) ) ;
#18791=LINE ( 'NONE', #2504, #15074 ) ;
#18796=EDGE_CURVE ( 'NONE', #8886, #15578, #2695, .T. ) ;
#18799=ADVANCED_BREP_SHAPE_REPRESENTATION ( '', ( #16536, #1791 ), #11098 ) ;
#18826=CARTESIAN_POINT ( 'NONE',  ( -7.499999999999994671, -38.00000000000000000, 4.500000000000000888 ) ) ;
#18837=EDGE_LOOP ( 'NONE', ( #18011, #11783, #6181, #556 ) ) ;
#18898=ORIENTED_EDGE ( 'NONE', *, *, #4029, .T. ) ;
#18902=ORIENTED_EDGE ( 'NONE', *, *, #18796, .F. ) ;
#18959=LINE ( 'NONE', #19156, #145 ) ;
#19156=CARTESIAN_POINT ( 'NONE',  ( -7.499999999999994671, -38.00000000000000000, 1.500000000000000000 ) ) ;
#19185=ORIENTED_EDGE ( 'NONE', *, *, #11905, .T. ) ;
#19275=AXIS2_PLACEMENT_3D ( 'NONE', #7424, #14877, #12023 ) ;
#19280=DIRECTION ( 'NONE',  ( 1.000000000000000000, 2.312964634635742957E-16, 0.000000000000000000 ) ) ;
#19315=ORIENTED_EDGE ( 'NONE', *, *, #1761, .T. ) ;
#19376=PLANE ( 'NONE',  #10660 ) ;
#19391=ORIENTED_EDGE ( 'NONE', *, *, #10310, .F. ) ;
ENDSEC;
END-ISO-10303-21;
